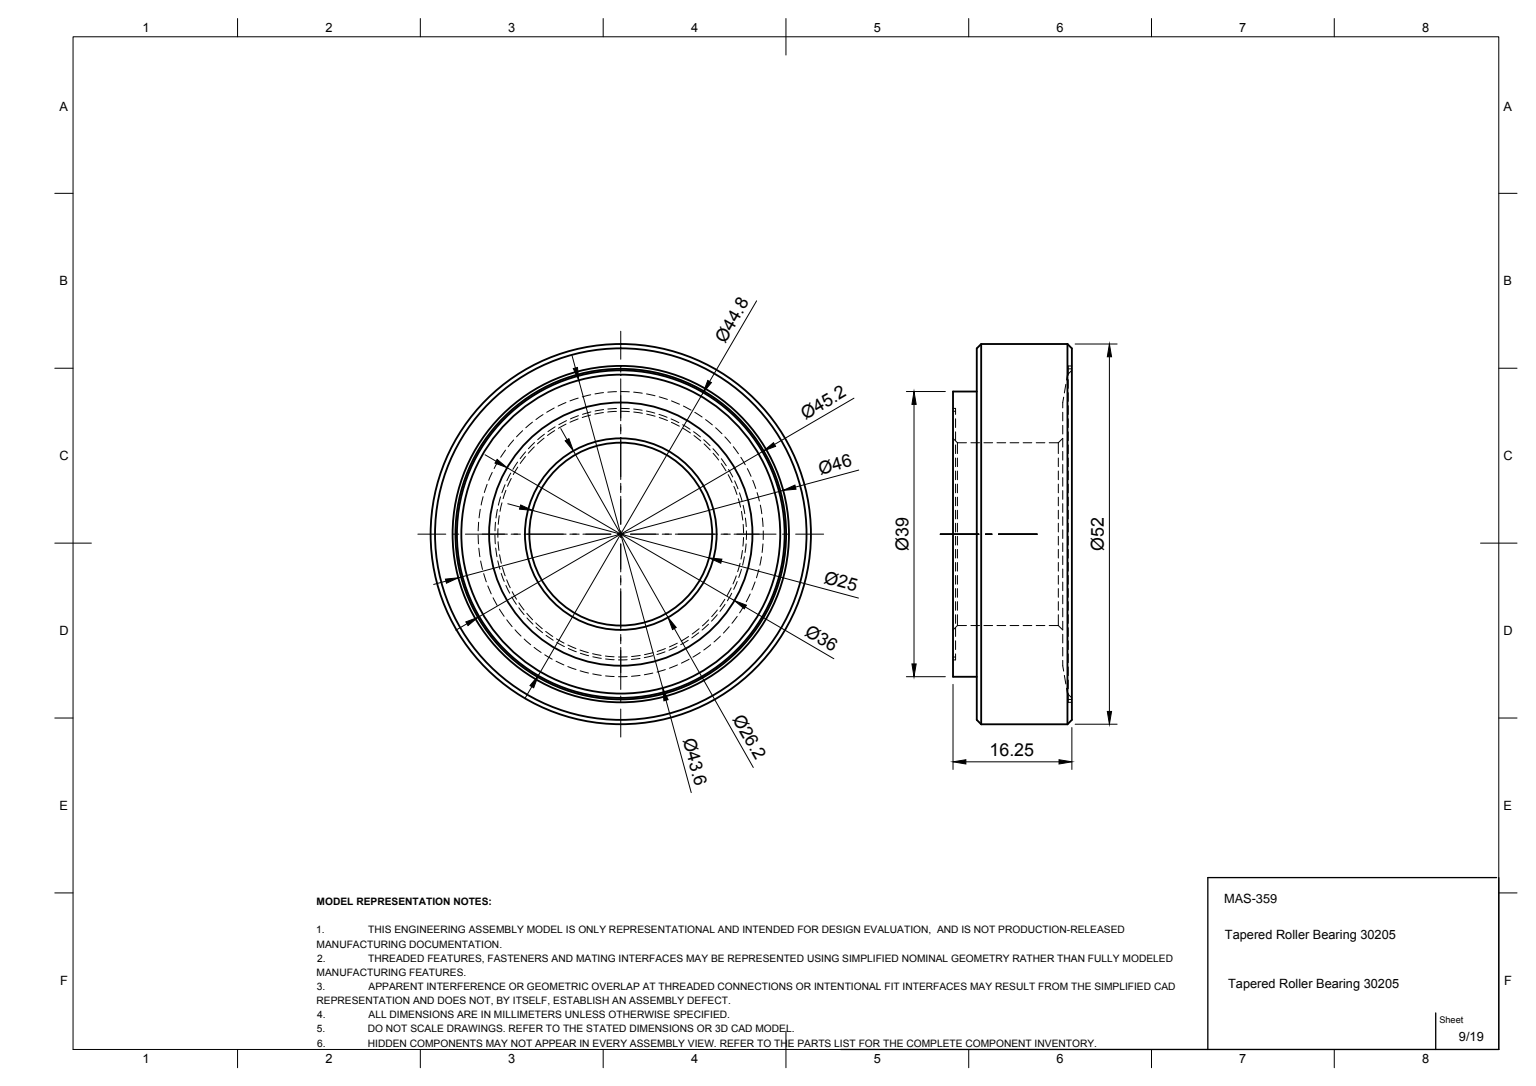
ISO-10303-21;
HEADER;
/* Generated by software containing ST-Developer
 * from STEP Tools, Inc. (www.steptools.com) 
 */

FILE_DESCRIPTION(
/* description */ (''),
/* implementation_level */ '2;1');

FILE_NAME(
/* name */ 'Tapered Roller Bearing 30205.step',
/* time_stamp */ '2026-10-15T14:25:16-07:00',
/* author */ (''),
/* organization */ (''),
/* preprocessor_version */ 'ST-DEVELOPER v20.2',
/* originating_system */ 'Autodesk Translation Framework v15.15.0.0',
/* authorisation */ '');

FILE_SCHEMA (('AUTOMOTIVE_DESIGN { 1 0 10303 214 3 1 1 }'));
ENDSEC;

DATA;
#10=MECHANICAL_DESIGN_GEOMETRIC_PRESENTATION_REPRESENTATION('',(#334),#86429);
#298=SHAPE_REPRESENTATION_RELATIONSHIP('SRR','None',#86513,#316);
#316=ADVANCED_BREP_SHAPE_REPRESENTATION('',(#352),#86422);
#334=STYLED_ITEM('',(#86612),#352);
#352=MANIFOLD_SOLID_BREP('Body1',#15624);
#1321=CONICAL_SURFACE('',#17007,1.28,0.785398163397449);
#1322=CONICAL_SURFACE('',#17011,1.99,1.40138328290528);
#1323=CONICAL_SURFACE('',#17013,2.21,0.785398163397445);
#1324=CONICAL_SURFACE('',#17016,2.57,0.785398163397449);
#1325=CONICAL_SURFACE('',#17020,2.57,0.785398163397448);
#1326=CONICAL_SURFACE('',#17027,1.28,0.785398163397448);
#1535=CYLINDRICAL_SURFACE('',#16986,2.26);
#1536=CYLINDRICAL_SURFACE('',#16989,2.3);
#1537=CYLINDRICAL_SURFACE('',#16993,1.68);
#1538=CYLINDRICAL_SURFACE('',#16998,1.72);
#1539=CYLINDRICAL_SURFACE('',#17004,1.25);
#1540=CYLINDRICAL_SURFACE('',#17018,2.6);
#1541=CYLINDRICAL_SURFACE('',#17024,1.95);
#1725=FACE_BOUND('',#4101,.T.);
#1726=FACE_BOUND('',#4104,.T.);
#1727=FACE_BOUND('',#4107,.T.);
#1728=FACE_BOUND('',#4109,.T.);
#1729=FACE_BOUND('',#4113,.T.);
#1730=FACE_BOUND('',#4117,.T.);
#1731=FACE_BOUND('',#4122,.T.);
#1732=FACE_BOUND('',#4125,.T.);
#2270=CIRCLE('',#16987,2.26);
#2271=CIRCLE('',#16988,2.26);
#2272=CIRCLE('',#16990,2.3);
#2273=CIRCLE('',#16991,2.3);
#2274=CIRCLE('',#16994,1.68);
#2275=CIRCLE('',#16995,1.68);
#2276=CIRCLE('',#16997,1.72);
#2277=CIRCLE('',#16999,1.72);
#2278=CIRCLE('',#17001,2.54);
#2279=CIRCLE('',#17003,1.95);
#2280=CIRCLE('',#17005,1.25);
#2281=CIRCLE('',#17006,1.25);
#2282=CIRCLE('',#17008,1.31);
#2283=CIRCLE('',#17010,1.8);
#2284=CIRCLE('',#17012,2.18);
#2285=CIRCLE('',#17014,2.24);
#2286=CIRCLE('',#17017,2.6);
#2287=CIRCLE('',#17019,2.6);
#2288=CIRCLE('',#17021,2.54);
#2289=CIRCLE('',#17023,1.95);
#2290=CIRCLE('',#17026,1.31);
#3103=FACE_OUTER_BOUND('',#4098,.T.);
#3104=FACE_OUTER_BOUND('',#4099,.T.);
#3105=FACE_OUTER_BOUND('',#4100,.T.);
#3106=FACE_OUTER_BOUND('',#4102,.T.);
#3107=FACE_OUTER_BOUND('',#4103,.T.);
#3108=FACE_OUTER_BOUND('',#4105,.T.);
#3109=FACE_OUTER_BOUND('',#4106,.T.);
#3110=FACE_OUTER_BOUND('',#4108,.T.);
#3111=FACE_OUTER_BOUND('',#4110,.T.);
#3112=FACE_OUTER_BOUND('',#4111,.T.);
#3113=FACE_OUTER_BOUND('',#4112,.T.);
#3114=FACE_OUTER_BOUND('',#4114,.T.);
#3115=FACE_OUTER_BOUND('',#4115,.T.);
#3116=FACE_OUTER_BOUND('',#4116,.T.);
#3117=FACE_OUTER_BOUND('',#4118,.T.);
#3118=FACE_OUTER_BOUND('',#4119,.T.);
#3119=FACE_OUTER_BOUND('',#4120,.T.);
#3120=FACE_OUTER_BOUND('',#4121,.T.);
#3121=FACE_OUTER_BOUND('',#4123,.T.);
#3122=FACE_OUTER_BOUND('',#4124,.T.);
#3123=FACE_OUTER_BOUND('',#4126,.T.);
#4098=EDGE_LOOP('',(#13559,#13560,#13561,#13562));
#4099=EDGE_LOOP('',(#13563,#13564,#13565,#13566));
#4100=EDGE_LOOP('',(#13567));
#4101=EDGE_LOOP('',(#13568));
#4102=EDGE_LOOP('',(#13569,#13570,#13571,#13572));
#4103=EDGE_LOOP('',(#13573));
#4104=EDGE_LOOP('',(#13574));
#4105=EDGE_LOOP('',(#13575,#13576,#13577,#13578));
#4106=EDGE_LOOP('',(#13579));
#4107=EDGE_LOOP('',(#13580));
#4108=EDGE_LOOP('',(#13581));
#4109=EDGE_LOOP('',(#13582));
#4110=EDGE_LOOP('',(#13583,#13584,#13585,#13586));
#4111=EDGE_LOOP('',(#13587,#13588,#13589,#13590));
#4112=EDGE_LOOP('',(#13591));
#4113=EDGE_LOOP('',(#13592));
#4114=EDGE_LOOP('',(#13593,#13594,#13595,#13596));
#4115=EDGE_LOOP('',(#13597,#13598,#13599,#13600));
#4116=EDGE_LOOP('',(#13601));
#4117=EDGE_LOOP('',(#13602));
#4118=EDGE_LOOP('',(#13603,#13604,#13605,#13606));
#4119=EDGE_LOOP('',(#13607,#13608,#13609,#13610));
#4120=EDGE_LOOP('',(#13611,#13612,#13613,#13614));
#4121=EDGE_LOOP('',(#13615));
#4122=EDGE_LOOP('',(#13616));
#4123=EDGE_LOOP('',(#13617,#13618,#13619,#13620));
#4124=EDGE_LOOP('',(#13621));
#4125=EDGE_LOOP('',(#13622));
#4126=EDGE_LOOP('',(#13623,#13624,#13625,#13626));
#5018=LINE('',#66378,#5878);
#5019=LINE('',#66384,#5879);
#5020=LINE('',#66391,#5880);
#5021=LINE('',#66398,#5881);
#5022=LINE('',#66410,#5882);
#5023=LINE('',#66414,#5883);
#5024=LINE('',#66421,#5884);
#5025=LINE('',#66425,#5885);
#5026=LINE('',#66431,#5886);
#5027=LINE('',#66435,#5887);
#5028=LINE('',#66438,#5888);
#5029=LINE('',#66444,#5889);
#5030=LINE('',#66449,#5890);
#5878=VECTOR('',#20339,2.26);
#5879=VECTOR('',#20346,2.3);
#5880=VECTOR('',#20355,1.68);
#5881=VECTOR('',#20364,1.72);
#5882=VECTOR('',#20379,1.25);
#5883=VECTOR('',#20384,1.28);
#5884=VECTOR('',#20393,1.99);
#5885=VECTOR('',#20398,2.21);
#5886=VECTOR('',#20407,2.57);
#5887=VECTOR('',#20412,2.6);
#5888=VECTOR('',#20415,2.57);
#5889=VECTOR('',#20424,1.95);
#5890=VECTOR('',#20431,1.28);
#7218=VERTEX_POINT('',#66375);
#7219=VERTEX_POINT('',#66377);
#7220=VERTEX_POINT('',#66381);
#7221=VERTEX_POINT('',#66383);
#7222=VERTEX_POINT('',#66388);
#7223=VERTEX_POINT('',#66390);
#7224=VERTEX_POINT('',#66394);
#7225=VERTEX_POINT('',#66397);
#7226=VERTEX_POINT('',#66401);
#7227=VERTEX_POINT('',#66404);
#7228=VERTEX_POINT('',#66407);
#7229=VERTEX_POINT('',#66409);
#7230=VERTEX_POINT('',#66413);
#7231=VERTEX_POINT('',#66417);
#7232=VERTEX_POINT('',#66420);
#7233=VERTEX_POINT('',#66424);
#7234=VERTEX_POINT('',#66429);
#7235=VERTEX_POINT('',#66433);
#7236=VERTEX_POINT('',#66437);
#7237=VERTEX_POINT('',#66441);
#7238=VERTEX_POINT('',#66446);
#9401=EDGE_CURVE('',#7218,#7218,#2270,.T.);
#9402=EDGE_CURVE('',#7218,#7219,#5018,.T.);
#9403=EDGE_CURVE('',#7219,#7219,#2271,.T.);
#9404=EDGE_CURVE('',#7220,#7220,#2272,.T.);
#9405=EDGE_CURVE('',#7220,#7221,#5019,.T.);
#9406=EDGE_CURVE('',#7221,#7221,#2273,.T.);
#9407=EDGE_CURVE('',#7222,#7222,#2274,.T.);
#9408=EDGE_CURVE('',#7222,#7223,#5020,.T.);
#9409=EDGE_CURVE('',#7223,#7223,#2275,.T.);
#9410=EDGE_CURVE('',#7224,#7224,#2276,.T.);
#9411=EDGE_CURVE('',#7224,#7225,#5021,.T.);
#9412=EDGE_CURVE('',#7225,#7225,#2277,.T.);
#9413=EDGE_CURVE('',#7226,#7226,#2278,.T.);
#9414=EDGE_CURVE('',#7227,#7227,#2279,.T.);
#9415=EDGE_CURVE('',#7228,#7228,#2280,.T.);
#9416=EDGE_CURVE('',#7228,#7229,#5022,.T.);
#9417=EDGE_CURVE('',#7229,#7229,#2281,.T.);
#9418=EDGE_CURVE('',#7228,#7230,#5023,.T.);
#9419=EDGE_CURVE('',#7230,#7230,#2282,.T.);
#9420=EDGE_CURVE('',#7231,#7231,#2283,.T.);
#9421=EDGE_CURVE('',#7231,#7232,#5024,.T.);
#9422=EDGE_CURVE('',#7232,#7232,#2284,.T.);
#9423=EDGE_CURVE('',#7232,#7233,#5025,.T.);
#9424=EDGE_CURVE('',#7233,#7233,#2285,.T.);
#9425=EDGE_CURVE('',#7234,#7234,#2286,.T.);
#9426=EDGE_CURVE('',#7234,#7226,#5026,.T.);
#9427=EDGE_CURVE('',#7235,#7235,#2287,.T.);
#9428=EDGE_CURVE('',#7235,#7234,#5027,.T.);
#9429=EDGE_CURVE('',#7235,#7236,#5028,.T.);
#9430=EDGE_CURVE('',#7236,#7236,#2288,.T.);
#9431=EDGE_CURVE('',#7237,#7237,#2289,.T.);
#9432=EDGE_CURVE('',#7227,#7237,#5029,.T.);
#9433=EDGE_CURVE('',#7238,#7238,#2290,.T.);
#9434=EDGE_CURVE('',#7229,#7238,#5030,.T.);
#13559=ORIENTED_EDGE('',*,*,#9401,.F.);
#13560=ORIENTED_EDGE('',*,*,#9402,.T.);
#13561=ORIENTED_EDGE('',*,*,#9403,.F.);
#13562=ORIENTED_EDGE('',*,*,#9402,.F.);
#13563=ORIENTED_EDGE('',*,*,#9404,.F.);
#13564=ORIENTED_EDGE('',*,*,#9405,.T.);
#13565=ORIENTED_EDGE('',*,*,#9406,.T.);
#13566=ORIENTED_EDGE('',*,*,#9405,.F.);
#13567=ORIENTED_EDGE('',*,*,#9406,.F.);
#13568=ORIENTED_EDGE('',*,*,#9401,.T.);
#13569=ORIENTED_EDGE('',*,*,#9407,.F.);
#13570=ORIENTED_EDGE('',*,*,#9408,.T.);
#13571=ORIENTED_EDGE('',*,*,#9409,.T.);
#13572=ORIENTED_EDGE('',*,*,#9408,.F.);
#13573=ORIENTED_EDGE('',*,*,#9410,.T.);
#13574=ORIENTED_EDGE('',*,*,#9409,.F.);
#13575=ORIENTED_EDGE('',*,*,#9410,.F.);
#13576=ORIENTED_EDGE('',*,*,#9411,.T.);
#13577=ORIENTED_EDGE('',*,*,#9412,.F.);
#13578=ORIENTED_EDGE('',*,*,#9411,.F.);
#13579=ORIENTED_EDGE('',*,*,#9413,.F.);
#13580=ORIENTED_EDGE('',*,*,#9404,.T.);
#13581=ORIENTED_EDGE('',*,*,#9414,.T.);
#13582=ORIENTED_EDGE('',*,*,#9412,.T.);
#13583=ORIENTED_EDGE('',*,*,#9415,.F.);
#13584=ORIENTED_EDGE('',*,*,#9416,.T.);
#13585=ORIENTED_EDGE('',*,*,#9417,.T.);
#13586=ORIENTED_EDGE('',*,*,#9416,.F.);
#13587=ORIENTED_EDGE('',*,*,#9415,.T.);
#13588=ORIENTED_EDGE('',*,*,#9418,.T.);
#13589=ORIENTED_EDGE('',*,*,#9419,.F.);
#13590=ORIENTED_EDGE('',*,*,#9418,.F.);
#13591=ORIENTED_EDGE('',*,*,#9420,.F.);
#13592=ORIENTED_EDGE('',*,*,#9419,.T.);
#13593=ORIENTED_EDGE('',*,*,#9420,.T.);
#13594=ORIENTED_EDGE('',*,*,#9421,.T.);
#13595=ORIENTED_EDGE('',*,*,#9422,.F.);
#13596=ORIENTED_EDGE('',*,*,#9421,.F.);
#13597=ORIENTED_EDGE('',*,*,#9422,.T.);
#13598=ORIENTED_EDGE('',*,*,#9423,.T.);
#13599=ORIENTED_EDGE('',*,*,#9424,.F.);
#13600=ORIENTED_EDGE('',*,*,#9423,.F.);
#13601=ORIENTED_EDGE('',*,*,#9403,.T.);
#13602=ORIENTED_EDGE('',*,*,#9424,.T.);
#13603=ORIENTED_EDGE('',*,*,#9425,.F.);
#13604=ORIENTED_EDGE('',*,*,#9426,.T.);
#13605=ORIENTED_EDGE('',*,*,#9413,.T.);
#13606=ORIENTED_EDGE('',*,*,#9426,.F.);
#13607=ORIENTED_EDGE('',*,*,#9427,.F.);
#13608=ORIENTED_EDGE('',*,*,#9428,.T.);
#13609=ORIENTED_EDGE('',*,*,#9425,.T.);
#13610=ORIENTED_EDGE('',*,*,#9428,.F.);
#13611=ORIENTED_EDGE('',*,*,#9427,.T.);
#13612=ORIENTED_EDGE('',*,*,#9429,.T.);
#13613=ORIENTED_EDGE('',*,*,#9430,.F.);
#13614=ORIENTED_EDGE('',*,*,#9429,.F.);
#13615=ORIENTED_EDGE('',*,*,#9430,.T.);
#13616=ORIENTED_EDGE('',*,*,#9431,.F.);
#13617=ORIENTED_EDGE('',*,*,#9414,.F.);
#13618=ORIENTED_EDGE('',*,*,#9432,.T.);
#13619=ORIENTED_EDGE('',*,*,#9431,.T.);
#13620=ORIENTED_EDGE('',*,*,#9432,.F.);
#13621=ORIENTED_EDGE('',*,*,#9407,.T.);
#13622=ORIENTED_EDGE('',*,*,#9433,.F.);
#13623=ORIENTED_EDGE('',*,*,#9417,.F.);
#13624=ORIENTED_EDGE('',*,*,#9434,.T.);
#13625=ORIENTED_EDGE('',*,*,#9433,.T.);
#13626=ORIENTED_EDGE('',*,*,#9434,.F.);
#14692=PLANE('',#16992);
#14693=PLANE('',#16996);
#14694=PLANE('',#17000);
#14695=PLANE('',#17002);
#14696=PLANE('',#17009);
#14697=PLANE('',#17015);
#14698=PLANE('',#17022);
#14699=PLANE('',#17025);
#15459=ADVANCED_FACE('',(#3103),#1535,.T.);
#15460=ADVANCED_FACE('',(#3104),#1536,.F.);
#15461=ADVANCED_FACE('',(#3105,#1725),#14692,.F.);
#15462=ADVANCED_FACE('',(#3106),#1537,.T.);
#15463=ADVANCED_FACE('',(#3107,#1726),#14693,.F.);
#15464=ADVANCED_FACE('',(#3108),#1538,.F.);
#15465=ADVANCED_FACE('',(#3109,#1727),#14694,.T.);
#15466=ADVANCED_FACE('',(#3110,#1728),#14695,.T.);
#15467=ADVANCED_FACE('',(#3111),#1539,.F.);
#15468=ADVANCED_FACE('',(#3112),#1321,.F.);
#15469=ADVANCED_FACE('',(#3113,#1729),#14696,.T.);
#15470=ADVANCED_FACE('',(#3114),#1322,.F.);
#15471=ADVANCED_FACE('',(#3115),#1323,.F.);
#15472=ADVANCED_FACE('',(#3116,#1730),#14697,.T.);
#15473=ADVANCED_FACE('',(#3117),#1324,.T.);
#15474=ADVANCED_FACE('',(#3118),#1540,.T.);
#15475=ADVANCED_FACE('',(#3119),#1325,.T.);
#15476=ADVANCED_FACE('',(#3120,#1731),#14698,.T.);
#15477=ADVANCED_FACE('',(#3121),#1541,.T.);
#15478=ADVANCED_FACE('',(#3122,#1732),#14699,.T.);
#15479=ADVANCED_FACE('',(#3123),#1326,.F.);
#15624=CLOSED_SHELL('',(#15459,#15460,#15461,#15462,#15463,#15464,#15465,
#15466,#15467,#15468,#15469,#15470,#15471,#15472,#15473,#15474,#15475,#15476,
#15477,#15478,#15479));
#16985=AXIS2_PLACEMENT_3D('',#66373,#20333,#20334);
#16986=AXIS2_PLACEMENT_3D('',#66374,#20335,#20336);
#16987=AXIS2_PLACEMENT_3D('',#66376,#20337,#20338);
#16988=AXIS2_PLACEMENT_3D('',#66379,#20340,#20341);
#16989=AXIS2_PLACEMENT_3D('',#66380,#20342,#20343);
#16990=AXIS2_PLACEMENT_3D('',#66382,#20344,#20345);
#16991=AXIS2_PLACEMENT_3D('',#66385,#20347,#20348);
#16992=AXIS2_PLACEMENT_3D('',#66386,#20349,#20350);
#16993=AXIS2_PLACEMENT_3D('',#66387,#20351,#20352);
#16994=AXIS2_PLACEMENT_3D('',#66389,#20353,#20354);
#16995=AXIS2_PLACEMENT_3D('',#66392,#20356,#20357);
#16996=AXIS2_PLACEMENT_3D('',#66393,#20358,#20359);
#16997=AXIS2_PLACEMENT_3D('',#66395,#20360,#20361);
#16998=AXIS2_PLACEMENT_3D('',#66396,#20362,#20363);
#16999=AXIS2_PLACEMENT_3D('',#66399,#20365,#20366);
#17000=AXIS2_PLACEMENT_3D('',#66400,#20367,#20368);
#17001=AXIS2_PLACEMENT_3D('',#66402,#20369,#20370);
#17002=AXIS2_PLACEMENT_3D('',#66403,#20371,#20372);
#17003=AXIS2_PLACEMENT_3D('',#66405,#20373,#20374);
#17004=AXIS2_PLACEMENT_3D('',#66406,#20375,#20376);
#17005=AXIS2_PLACEMENT_3D('',#66408,#20377,#20378);
#17006=AXIS2_PLACEMENT_3D('',#66411,#20380,#20381);
#17007=AXIS2_PLACEMENT_3D('',#66412,#20382,#20383);
#17008=AXIS2_PLACEMENT_3D('',#66415,#20385,#20386);
#17009=AXIS2_PLACEMENT_3D('',#66416,#20387,#20388);
#17010=AXIS2_PLACEMENT_3D('',#66418,#20389,#20390);
#17011=AXIS2_PLACEMENT_3D('',#66419,#20391,#20392);
#17012=AXIS2_PLACEMENT_3D('',#66422,#20394,#20395);
#17013=AXIS2_PLACEMENT_3D('',#66423,#20396,#20397);
#17014=AXIS2_PLACEMENT_3D('',#66426,#20399,#20400);
#17015=AXIS2_PLACEMENT_3D('',#66427,#20401,#20402);
#17016=AXIS2_PLACEMENT_3D('',#66428,#20403,#20404);
#17017=AXIS2_PLACEMENT_3D('',#66430,#20405,#20406);
#17018=AXIS2_PLACEMENT_3D('',#66432,#20408,#20409);
#17019=AXIS2_PLACEMENT_3D('',#66434,#20410,#20411);
#17020=AXIS2_PLACEMENT_3D('',#66436,#20413,#20414);
#17021=AXIS2_PLACEMENT_3D('',#66439,#20416,#20417);
#17022=AXIS2_PLACEMENT_3D('',#66440,#20418,#20419);
#17023=AXIS2_PLACEMENT_3D('',#66442,#20420,#20421);
#17024=AXIS2_PLACEMENT_3D('',#66443,#20422,#20423);
#17025=AXIS2_PLACEMENT_3D('',#66445,#20425,#20426);
#17026=AXIS2_PLACEMENT_3D('',#66447,#20427,#20428);
#17027=AXIS2_PLACEMENT_3D('',#66448,#20429,#20430);
#20333=DIRECTION('axis',(0.,0.,1.));
#20334=DIRECTION('refdir',(1.,0.,0.));
#20335=DIRECTION('center_axis',(0.,0.,1.));
#20336=DIRECTION('ref_axis',(1.,0.,0.));
#20337=DIRECTION('center_axis',(0.,0.,1.));
#20338=DIRECTION('ref_axis',(1.,0.,0.));
#20339=DIRECTION('',(0.,0.,-1.));
#20340=DIRECTION('center_axis',(0.,0.,-1.));
#20341=DIRECTION('ref_axis',(1.,0.,0.));
#20342=DIRECTION('center_axis',(0.,0.,1.));
#20343=DIRECTION('ref_axis',(1.,0.,0.));
#20344=DIRECTION('center_axis',(0.,0.,1.));
#20345=DIRECTION('ref_axis',(1.,0.,0.));
#20346=DIRECTION('',(0.,0.,1.));
#20347=DIRECTION('center_axis',(0.,0.,1.));
#20348=DIRECTION('ref_axis',(1.,0.,0.));
#20349=DIRECTION('center_axis',(0.,0.,1.));
#20350=DIRECTION('ref_axis',(1.,0.,0.));
#20351=DIRECTION('center_axis',(0.,0.,1.));
#20352=DIRECTION('ref_axis',(1.,0.,0.));
#20353=DIRECTION('center_axis',(0.,0.,1.));
#20354=DIRECTION('ref_axis',(1.,0.,0.));
#20355=DIRECTION('',(0.,0.,-1.));
#20356=DIRECTION('center_axis',(0.,0.,1.));
#20357=DIRECTION('ref_axis',(1.,0.,0.));
#20358=DIRECTION('center_axis',(0.,0.,-1.));
#20359=DIRECTION('ref_axis',(-1.,0.,0.));
#20360=DIRECTION('center_axis',(0.,0.,1.));
#20361=DIRECTION('ref_axis',(1.,0.,0.));
#20362=DIRECTION('center_axis',(0.,0.,1.));
#20363=DIRECTION('ref_axis',(1.,0.,0.));
#20364=DIRECTION('',(0.,0.,1.));
#20365=DIRECTION('center_axis',(0.,0.,-1.));
#20366=DIRECTION('ref_axis',(1.,0.,0.));
#20367=DIRECTION('center_axis',(0.,0.,-1.));
#20368=DIRECTION('ref_axis',(-1.,0.,0.));
#20369=DIRECTION('center_axis',(0.,0.,1.));
#20370=DIRECTION('ref_axis',(1.,0.,0.));
#20371=DIRECTION('center_axis',(0.,0.,1.));
#20372=DIRECTION('ref_axis',(1.,0.,0.));
#20373=DIRECTION('center_axis',(0.,0.,1.));
#20374=DIRECTION('ref_axis',(1.,0.,0.));
#20375=DIRECTION('center_axis',(0.,0.,1.));
#20376=DIRECTION('ref_axis',(1.,0.,0.));
#20377=DIRECTION('center_axis',(0.,0.,1.));
#20378=DIRECTION('ref_axis',(1.,0.,0.));
#20379=DIRECTION('',(0.,0.,1.));
#20380=DIRECTION('center_axis',(0.,0.,1.));
#20381=DIRECTION('ref_axis',(1.,0.,0.));
#20382=DIRECTION('center_axis',(0.,0.,-1.));
#20383=DIRECTION('ref_axis',(1.,0.,0.));
#20384=DIRECTION('',(-0.707106781186548,8.65956056235494E-17,-0.707106781186547));
#20385=DIRECTION('center_axis',(0.,0.,1.));
#20386=DIRECTION('ref_axis',(1.,0.,0.));
#20387=DIRECTION('center_axis',(0.,0.,-1.));
#20388=DIRECTION('ref_axis',(-1.,0.,0.));
#20389=DIRECTION('center_axis',(0.,0.,1.));
#20390=DIRECTION('ref_axis',(1.,0.,0.));
#20391=DIRECTION('center_axis',(0.,0.,-1.));
#20392=DIRECTION('ref_axis',(1.,0.,0.));
#20393=DIRECTION('',(-0.98568389974183,1.20711463278991E-16,-0.168603824955838));
#20394=DIRECTION('center_axis',(0.,0.,1.));
#20395=DIRECTION('ref_axis',(1.,0.,0.));
#20396=DIRECTION('center_axis',(0.,0.,-1.));
#20397=DIRECTION('ref_axis',(1.,0.,0.));
#20398=DIRECTION('',(-0.707106781186545,8.6595605623549E-17,-0.70710678118655));
#20399=DIRECTION('center_axis',(0.,0.,1.));
#20400=DIRECTION('ref_axis',(1.,0.,0.));
#20401=DIRECTION('center_axis',(0.,0.,-1.));
#20402=DIRECTION('ref_axis',(-1.,0.,0.));
#20403=DIRECTION('center_axis',(0.,0.,1.));
#20404=DIRECTION('ref_axis',(1.,0.,0.));
#20405=DIRECTION('center_axis',(0.,0.,1.));
#20406=DIRECTION('ref_axis',(1.,0.,0.));
#20407=DIRECTION('',(0.707106781186548,8.65956056235494E-17,-0.707106781186547));
#20408=DIRECTION('center_axis',(0.,0.,1.));
#20409=DIRECTION('ref_axis',(1.,0.,0.));
#20410=DIRECTION('center_axis',(0.,0.,1.));
#20411=DIRECTION('ref_axis',(1.,0.,0.));
#20412=DIRECTION('',(0.,0.,-1.));
#20413=DIRECTION('center_axis',(0.,0.,-1.));
#20414=DIRECTION('ref_axis',(1.,0.,0.));
#20415=DIRECTION('',(0.707106781186547,-8.65956056235493E-17,0.707106781186548));
#20416=DIRECTION('center_axis',(0.,0.,1.));
#20417=DIRECTION('ref_axis',(1.,0.,0.));
#20418=DIRECTION('center_axis',(0.,0.,1.));
#20419=DIRECTION('ref_axis',(1.,0.,0.));
#20420=DIRECTION('center_axis',(0.,0.,1.));
#20421=DIRECTION('ref_axis',(1.,0.,0.));
#20422=DIRECTION('center_axis',(0.,0.,1.));
#20423=DIRECTION('ref_axis',(1.,0.,0.));
#20424=DIRECTION('',(0.,0.,-1.));
#20425=DIRECTION('center_axis',(0.,0.,1.));
#20426=DIRECTION('ref_axis',(1.,0.,0.));
#20427=DIRECTION('center_axis',(0.,0.,1.));
#20428=DIRECTION('ref_axis',(1.,0.,0.));
#20429=DIRECTION('center_axis',(0.,0.,1.));
#20430=DIRECTION('ref_axis',(1.,0.,0.));
#20431=DIRECTION('',(-0.707106781186547,-8.65956056235493E-17,0.707106781186548));
#66373=CARTESIAN_POINT('',(0.,0.,0.));
#66374=CARTESIAN_POINT('Origin',(0.,0.,0.02));
#66375=CARTESIAN_POINT('',(-2.26,-2.76770176607302E-16,0.05));
#66376=CARTESIAN_POINT('Origin',(0.,0.,0.05));
#66377=CARTESIAN_POINT('',(-2.26,2.76770176607302E-16,0.));
#66378=CARTESIAN_POINT('',(-2.26,-2.76770176607302E-16,0.02));
#66379=CARTESIAN_POINT('Origin',(0.,0.,0.));
#66380=CARTESIAN_POINT('Origin',(0.,0.,0.02));
#66381=CARTESIAN_POINT('',(-2.3,-2.81668763803891E-16,0.));
#66382=CARTESIAN_POINT('Origin',(0.,0.,0.));
#66383=CARTESIAN_POINT('',(-2.3,-2.81668763803891E-16,0.05));
#66384=CARTESIAN_POINT('',(-2.3,-2.81668763803891E-16,0.02));
#66385=CARTESIAN_POINT('Origin',(0.,0.,0.05));
#66386=CARTESIAN_POINT('Origin',(2.26,0.,0.05));
#66387=CARTESIAN_POINT('Origin',(0.,0.,1.615));
#66388=CARTESIAN_POINT('',(-1.68,-2.05740662256755E-16,1.625));
#66389=CARTESIAN_POINT('Origin',(0.,0.,1.625));
#66390=CARTESIAN_POINT('',(-1.68,-2.05740662256755E-16,1.59));
#66391=CARTESIAN_POINT('',(-1.68,-2.05740662256755E-16,1.615));
#66392=CARTESIAN_POINT('Origin',(0.,0.,1.59));
#66393=CARTESIAN_POINT('Origin',(1.72,0.,1.59));
#66394=CARTESIAN_POINT('',(-1.72,-2.10639249453345E-16,1.59));
#66395=CARTESIAN_POINT('Origin',(0.,0.,1.59));
#66396=CARTESIAN_POINT('Origin',(0.,0.,1.615));
#66397=CARTESIAN_POINT('',(-1.72,2.10639249453345E-16,1.625));
#66398=CARTESIAN_POINT('',(-1.72,-2.10639249453345E-16,1.615));
#66399=CARTESIAN_POINT('Origin',(0.,0.,1.625));
#66400=CARTESIAN_POINT('Origin',(2.54,0.,0.));
#66401=CARTESIAN_POINT('',(-2.54,-3.11060286983428E-16,-9.71445146547012E-17));
#66402=CARTESIAN_POINT('Origin',(0.,0.,0.));
#66403=CARTESIAN_POINT('Origin',(1.31,0.,1.625));
#66404=CARTESIAN_POINT('',(-1.95,-2.38806125833734E-16,1.625));
#66405=CARTESIAN_POINT('Origin',(0.,0.,1.625));
#66406=CARTESIAN_POINT('Origin',(0.,0.,0.875));
#66407=CARTESIAN_POINT('',(-1.25,-1.53080849893419E-16,0.185));
#66408=CARTESIAN_POINT('Origin',(0.,0.,0.185));
#66409=CARTESIAN_POINT('',(-1.25,-1.53080849893419E-16,1.565));
#66410=CARTESIAN_POINT('',(-1.25,-1.53080849893419E-16,0.875));
#66411=CARTESIAN_POINT('Origin',(0.,0.,1.565));
#66412=CARTESIAN_POINT('Origin',(0.,0.,0.155));
#66413=CARTESIAN_POINT('',(-1.31,-1.60428730688303E-16,0.125));
#66414=CARTESIAN_POINT('',(-1.28,1.56754790290861E-16,0.155));
#66415=CARTESIAN_POINT('Origin',(0.,0.,0.125));
#66416=CARTESIAN_POINT('Origin',(1.8,0.,0.125));
#66417=CARTESIAN_POINT('',(-1.8,-2.20436423846524E-16,0.125));
#66418=CARTESIAN_POINT('Origin',(0.,0.,0.125));
#66419=CARTESIAN_POINT('Origin',(0.,0.,0.0925));
#66420=CARTESIAN_POINT('',(-2.18,-2.66973002214123E-16,0.06));
#66421=CARTESIAN_POINT('',(-1.99,2.43704713030323E-16,0.0925));
#66422=CARTESIAN_POINT('Origin',(0.,0.,0.0600000000000001));
#66423=CARTESIAN_POINT('Origin',(0.,0.,0.03));
#66424=CARTESIAN_POINT('',(-2.24,-2.74320883009007E-16,1.73472347597681E-17));
#66425=CARTESIAN_POINT('',(-2.21,2.70646942611565E-16,0.03));
#66426=CARTESIAN_POINT('Origin',(0.,0.,0.));
#66427=CARTESIAN_POINT('Origin',(2.54,0.,0.));
#66428=CARTESIAN_POINT('Origin',(0.,0.,0.03));
#66429=CARTESIAN_POINT('',(-2.6,-3.18408167778312E-16,0.0599999999999999));
#66430=CARTESIAN_POINT('Origin',(0.,0.,0.0600000000000001));
#66431=CARTESIAN_POINT('',(-2.57,-3.1473422738087E-16,0.03));
#66432=CARTESIAN_POINT('Origin',(0.,0.,0.65));
#66433=CARTESIAN_POINT('',(-2.6,-3.18408167778312E-16,1.24));
#66434=CARTESIAN_POINT('Origin',(0.,0.,1.24));
#66435=CARTESIAN_POINT('',(-2.6,-3.18408167778312E-16,0.65));
#66436=CARTESIAN_POINT('Origin',(0.,0.,1.27));
#66437=CARTESIAN_POINT('',(-2.54,-3.11060286983428E-16,1.3));
#66438=CARTESIAN_POINT('',(-2.57,3.1473422738087E-16,1.27));
#66439=CARTESIAN_POINT('Origin',(0.,0.,1.3));
#66440=CARTESIAN_POINT('Origin',(1.95,0.,1.3));
#66441=CARTESIAN_POINT('',(-1.95,-2.38806125833734E-16,1.3));
#66442=CARTESIAN_POINT('Origin',(0.,0.,1.3));
#66443=CARTESIAN_POINT('Origin',(0.,0.,1.4625));
#66444=CARTESIAN_POINT('',(-1.95,-2.38806125833734E-16,1.4625));
#66445=CARTESIAN_POINT('Origin',(1.31,0.,1.625));
#66446=CARTESIAN_POINT('',(-1.31,-1.60428730688303E-16,1.625));
#66447=CARTESIAN_POINT('Origin',(0.,0.,1.625));
#66448=CARTESIAN_POINT('Origin',(0.,0.,1.595));
#66449=CARTESIAN_POINT('',(-1.28,-1.56754790290861E-16,1.595));
#86402=UNCERTAINTY_MEASURE_WITH_UNIT(LENGTH_MEASURE(0.001),#86430,
'DISTANCE_ACCURACY_VALUE',
'Maximum model space distance between geometric entities at asserted c
onnectivities');
#86409=UNCERTAINTY_MEASURE_WITH_UNIT(LENGTH_MEASURE(0.001),#86430,
'DISTANCE_ACCURACY_VALUE',
'Maximum model space distance between geometric entities at asserted c
onnectivities');
#86422=(
GEOMETRIC_REPRESENTATION_CONTEXT(3)
GLOBAL_UNCERTAINTY_ASSIGNED_CONTEXT((#86402))
GLOBAL_UNIT_ASSIGNED_CONTEXT((#86430,#86432,#86433))
REPRESENTATION_CONTEXT('','3D')
);
#86429=(
GEOMETRIC_REPRESENTATION_CONTEXT(3)
GLOBAL_UNCERTAINTY_ASSIGNED_CONTEXT((#86409))
GLOBAL_UNIT_ASSIGNED_CONTEXT((#86430,#86432,#86433))
REPRESENTATION_CONTEXT('','3D')
);
#86430=(
LENGTH_UNIT()
NAMED_UNIT(*)
SI_UNIT(.CENTI.,.METRE.)
);
#86432=(
NAMED_UNIT(*)
PLANE_ANGLE_UNIT()
SI_UNIT($,.RADIAN.)
);
#86433=(
NAMED_UNIT(*)
SI_UNIT($,.STERADIAN.)
SOLID_ANGLE_UNIT()
);
#86446=SHAPE_DEFINITION_REPRESENTATION(#86465,#86513);
#86465=PRODUCT_DEFINITION_SHAPE('',$,#86533);
#86513=SHAPE_REPRESENTATION('',(#16985),#86422);
#86520=PRODUCT_DEFINITION_CONTEXT('part definition',#86579,'design');
#86533=PRODUCT_DEFINITION('Tapered Roller Bearing 30205',
'Tapered Roller Bearing 30205',#86552,#86520);
#86552=PRODUCT_DEFINITION_FORMATION('',$,#86593);
#86579=APPLICATION_CONTEXT(
'Core Data for Automotive Mechanical Design Process');
#86580=PRODUCT_CONTEXT('part definition',#86579,'mechanical');
#86593=PRODUCT('Tapered Roller Bearing 30205',
'Tapered Roller Bearing 30205',$,(#86580));
#86612=PRESENTATION_STYLE_ASSIGNMENT((#86630));
#86630=SURFACE_STYLE_USAGE(.BOTH.,#86648);
#86648=SURFACE_SIDE_STYLE('',(#86666));
#86666=SURFACE_STYLE_FILL_AREA(#86684);
#86684=FILL_AREA_STYLE('Opaque(218,221,226)',(#86702));
#86702=FILL_AREA_STYLE_COLOUR('Opaque(218,221,226)',#86720);
#86720=COLOUR_RGB('Opaque(218,221,226)', 0.08235294, 0.09019608, 0.10196078);
ENDSEC;
END-ISO-10303-21;
